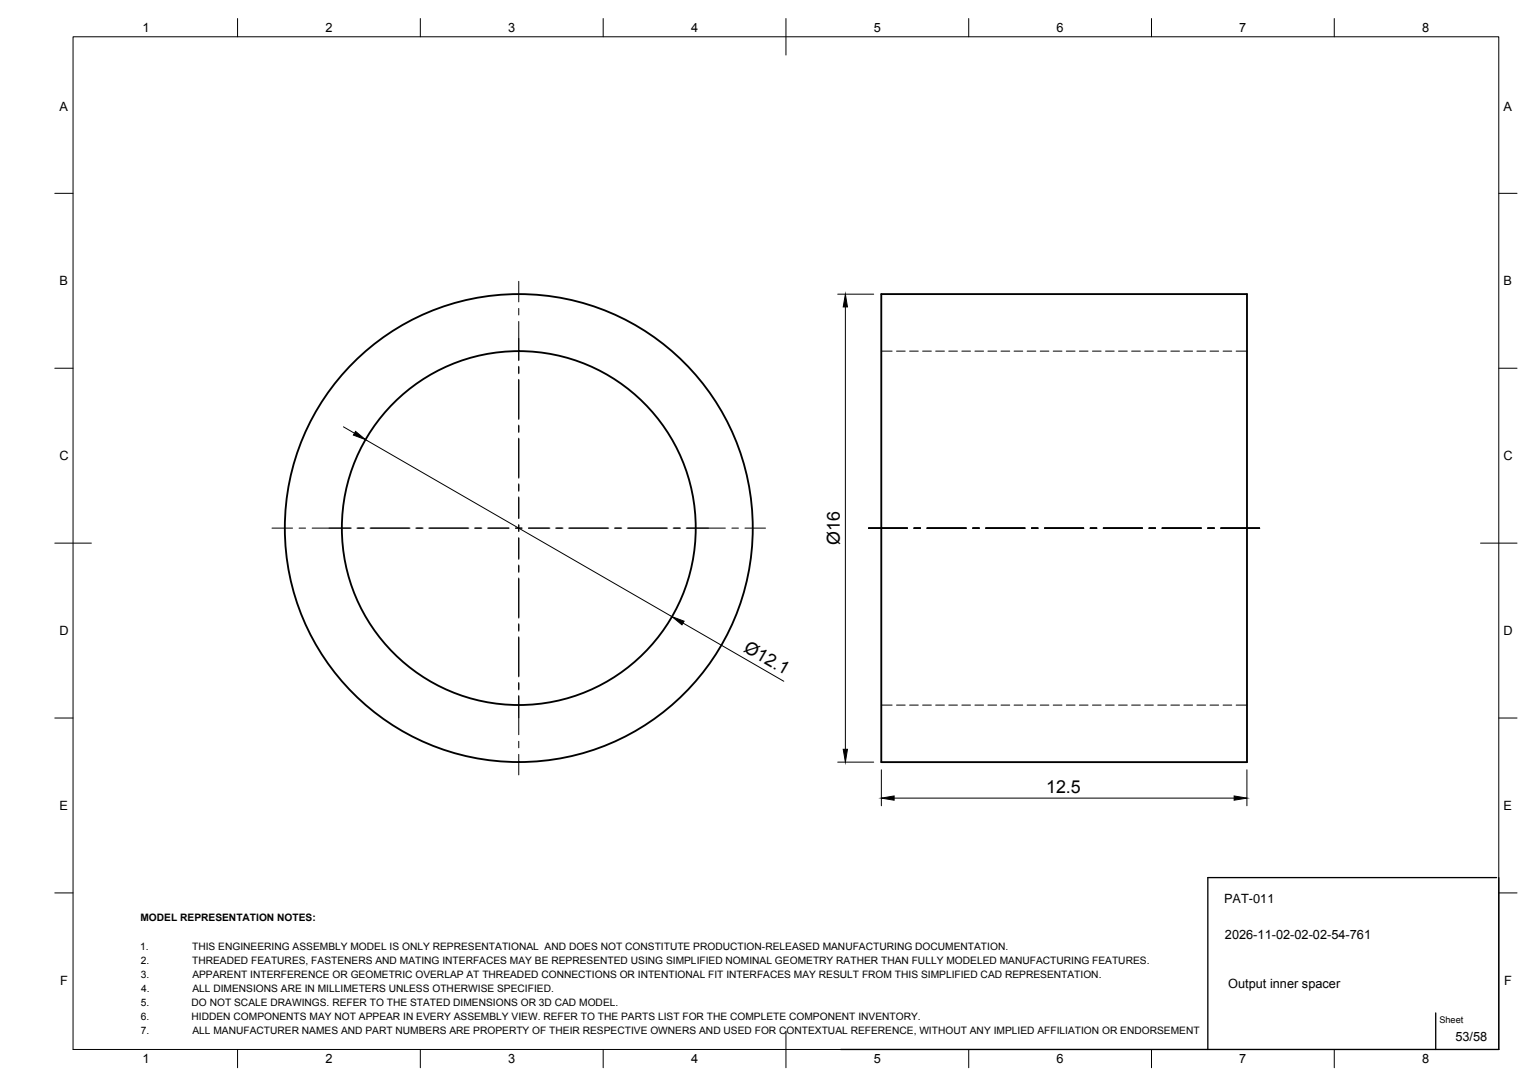
ISO-10303-21;
HEADER;
/* Generated by software containing ST-Developer
 * from STEP Tools, Inc. (www.steptools.com) 
 */

FILE_DESCRIPTION(
/* description */ ('Belt tension measurement rig'),
/* implementation_level */ '2;1');

FILE_NAME(
/* name */ 'Output inner spacer.step',
/* time_stamp */ '2026-10-28T03:24:44-07:00',
/* author */ (''),
/* organization */ (''),
/* preprocessor_version */ 'ST-DEVELOPER v20.2',
/* originating_system */ 'Autodesk Translation Framework v15.17.0.0',
/* authorisation */ '');

FILE_SCHEMA (('AUTOMOTIVE_DESIGN { 1 0 10303 214 3 1 1 }'));
ENDSEC;

DATA;
#10=MECHANICAL_DESIGN_GEOMETRIC_PRESENTATION_REPRESENTATION('',(#752),#23587);
#627=SHAPE_REPRESENTATION_RELATIONSHIP('SRR','None',#23878,#682);
#682=ADVANCED_BREP_SHAPE_REPRESENTATION('',(#820),#23576);
#752=STYLED_ITEM('',(#24204),#820);
#820=MANIFOLD_SOLID_BREP('Body1',#12259);
#1009=FACE_BOUND('',#2779,.T.);
#1010=FACE_BOUND('',#2781,.T.);
#1304=PLANE('',#14039);
#1305=PLANE('',#14040);
#1892=FACE_OUTER_BOUND('',#2776,.T.);
#1893=FACE_OUTER_BOUND('',#2777,.T.);
#1894=FACE_OUTER_BOUND('',#2778,.T.);
#1895=FACE_OUTER_BOUND('',#2780,.T.);
#2776=EDGE_LOOP('',(#10348,#10349,#10350,#10351));
#2777=EDGE_LOOP('',(#10352,#10353,#10354,#10355));
#2778=EDGE_LOOP('',(#10356));
#2779=EDGE_LOOP('',(#10357));
#2780=EDGE_LOOP('',(#10358));
#2781=EDGE_LOOP('',(#10359));
#3561=LINE('',#22187,#4312);
#3562=LINE('',#22193,#4313);
#4312=VECTOR('',#17428,0.605);
#4313=VECTOR('',#17435,0.800000000000001);
#5020=CIRCLE('',#14034,0.605);
#5021=CIRCLE('',#14035,0.605);
#5022=CIRCLE('',#14037,0.800000000000001);
#5023=CIRCLE('',#14038,0.800000000000001);
#6057=VERTEX_POINT('',#22184);
#6058=VERTEX_POINT('',#22186);
#6059=VERTEX_POINT('',#22190);
#6060=VERTEX_POINT('',#22192);
#7533=EDGE_CURVE('',#6057,#6057,#5020,.T.);
#7534=EDGE_CURVE('',#6057,#6058,#3561,.T.);
#7535=EDGE_CURVE('',#6058,#6058,#5021,.T.);
#7536=EDGE_CURVE('',#6059,#6059,#5022,.T.);
#7537=EDGE_CURVE('',#6059,#6060,#3562,.T.);
#7538=EDGE_CURVE('',#6060,#6060,#5023,.T.);
#10348=ORIENTED_EDGE('',*,*,#7533,.F.);
#10349=ORIENTED_EDGE('',*,*,#7534,.T.);
#10350=ORIENTED_EDGE('',*,*,#7535,.T.);
#10351=ORIENTED_EDGE('',*,*,#7534,.F.);
#10352=ORIENTED_EDGE('',*,*,#7536,.F.);
#10353=ORIENTED_EDGE('',*,*,#7537,.T.);
#10354=ORIENTED_EDGE('',*,*,#7538,.T.);
#10355=ORIENTED_EDGE('',*,*,#7537,.F.);
#10356=ORIENTED_EDGE('',*,*,#7536,.T.);
#10357=ORIENTED_EDGE('',*,*,#7533,.T.);
#10358=ORIENTED_EDGE('',*,*,#7538,.F.);
#10359=ORIENTED_EDGE('',*,*,#7535,.F.);
#11383=CYLINDRICAL_SURFACE('',#14033,0.605);
#11384=CYLINDRICAL_SURFACE('',#14036,0.800000000000001);
#12033=ADVANCED_FACE('',(#1892),#11383,.F.);
#12034=ADVANCED_FACE('',(#1893),#11384,.T.);
#12035=ADVANCED_FACE('',(#1894,#1009),#1304,.T.);
#12036=ADVANCED_FACE('',(#1895,#1010),#1305,.F.);
#12259=CLOSED_SHELL('',(#12033,#12034,#12035,#12036));
#14032=AXIS2_PLACEMENT_3D('',#22182,#17422,#17423);
#14033=AXIS2_PLACEMENT_3D('',#22183,#17424,#17425);
#14034=AXIS2_PLACEMENT_3D('',#22185,#17426,#17427);
#14035=AXIS2_PLACEMENT_3D('',#22188,#17429,#17430);
#14036=AXIS2_PLACEMENT_3D('',#22189,#17431,#17432);
#14037=AXIS2_PLACEMENT_3D('',#22191,#17433,#17434);
#14038=AXIS2_PLACEMENT_3D('',#22194,#17436,#17437);
#14039=AXIS2_PLACEMENT_3D('',#22195,#17438,#17439);
#14040=AXIS2_PLACEMENT_3D('',#22196,#17440,#17441);
#17422=DIRECTION('axis',(0.,0.,1.));
#17423=DIRECTION('refdir',(1.,0.,0.));
#17424=DIRECTION('center_axis',(0.,1.,0.));
#17425=DIRECTION('ref_axis',(1.,0.,0.));
#17426=DIRECTION('center_axis',(0.,-1.,0.));
#17427=DIRECTION('ref_axis',(1.,0.,0.));
#17428=DIRECTION('',(0.,-1.,0.));
#17429=DIRECTION('center_axis',(0.,-1.,0.));
#17430=DIRECTION('ref_axis',(1.,0.,0.));
#17431=DIRECTION('center_axis',(0.,1.,0.));
#17432=DIRECTION('ref_axis',(1.,0.,0.));
#17433=DIRECTION('center_axis',(0.,1.,0.));
#17434=DIRECTION('ref_axis',(1.,0.,0.));
#17435=DIRECTION('',(0.,-1.,0.));
#17436=DIRECTION('center_axis',(0.,1.,0.));
#17437=DIRECTION('ref_axis',(1.,0.,0.));
#17438=DIRECTION('center_axis',(0.,1.,0.));
#17439=DIRECTION('ref_axis',(1.,0.,0.));
#17440=DIRECTION('center_axis',(0.,1.,0.));
#17441=DIRECTION('ref_axis',(1.,0.,0.));
#22182=CARTESIAN_POINT('',(0.,0.,0.));
#22183=CARTESIAN_POINT('Origin',(10.,-2.65,7.));
#22184=CARTESIAN_POINT('',(9.395,-1.4,7.));
#22185=CARTESIAN_POINT('Origin',(10.,-1.4,7.));
#22186=CARTESIAN_POINT('',(9.395,-2.65,7.));
#22187=CARTESIAN_POINT('',(9.395,-2.65,7.));
#22188=CARTESIAN_POINT('Origin',(10.,-2.65,7.));
#22189=CARTESIAN_POINT('Origin',(10.,-2.65,7.));
#22190=CARTESIAN_POINT('',(9.2,-1.4,7.));
#22191=CARTESIAN_POINT('Origin',(10.,-1.4,7.));
#22192=CARTESIAN_POINT('',(9.2,-2.65,7.));
#22193=CARTESIAN_POINT('',(9.2,-2.65,7.));
#22194=CARTESIAN_POINT('Origin',(10.,-2.65,7.));
#22195=CARTESIAN_POINT('Origin',(10.,-1.4,7.));
#22196=CARTESIAN_POINT('Origin',(10.,-2.65,7.));
#23511=UNCERTAINTY_MEASURE_WITH_UNIT(LENGTH_MEASURE(0.001),#23588,
'DISTANCE_ACCURACY_VALUE',
'Maximum model space distance between geometric entities at asserted c
onnectivities');
#23522=UNCERTAINTY_MEASURE_WITH_UNIT(LENGTH_MEASURE(0.001),#23588,
'DISTANCE_ACCURACY_VALUE',
'Maximum model space distance between geometric entities at asserted c
onnectivities');
#23576=(
GEOMETRIC_REPRESENTATION_CONTEXT(3)
GLOBAL_UNCERTAINTY_ASSIGNED_CONTEXT((#23511))
GLOBAL_UNIT_ASSIGNED_CONTEXT((#23588,#23590,#23591))
REPRESENTATION_CONTEXT('','3D')
);
#23587=(
GEOMETRIC_REPRESENTATION_CONTEXT(3)
GLOBAL_UNCERTAINTY_ASSIGNED_CONTEXT((#23522))
GLOBAL_UNIT_ASSIGNED_CONTEXT((#23588,#23590,#23591))
REPRESENTATION_CONTEXT('','3D')
);
#23588=(
LENGTH_UNIT()
NAMED_UNIT(*)
SI_UNIT(.CENTI.,.METRE.)
);
#23590=(
NAMED_UNIT(*)
PLANE_ANGLE_UNIT()
SI_UNIT($,.RADIAN.)
);
#23591=(
NAMED_UNIT(*)
SI_UNIT($,.STERADIAN.)
SOLID_ANGLE_UNIT()
);
#23645=SHAPE_DEFINITION_REPRESENTATION(#23722,#23878);
#23722=PRODUCT_DEFINITION_SHAPE('',$,#23943);
#23878=SHAPE_REPRESENTATION('',(#14032),#23576);
#23889=PRODUCT_DEFINITION_CONTEXT('part definition',#24083,'design');
#23943=PRODUCT_DEFINITION('Output inner spacer','Output inner spacer',#24007,
#23889);
#24007=PRODUCT_DEFINITION_FORMATION('',$,#24138);
#24083=APPLICATION_CONTEXT(
'Core Data for Automotive Mechanical Design Process');
#24084=PRODUCT_CONTEXT('part definition',#24083,'mechanical');
#24138=PRODUCT('Output inner spacer','Output inner spacer',
'Output inner spacer',(#24084));
#24198=COLOUR_RGB('Sky Blue',0.24,0.69,0.87);
#24199=FILL_AREA_STYLE_COLOUR('',#24198);
#24200=FILL_AREA_STYLE('',(#24199));
#24201=SURFACE_STYLE_FILL_AREA(#24200);
#24202=SURFACE_SIDE_STYLE('',(#24201));
#24203=SURFACE_STYLE_USAGE(.BOTH.,#24202);
#24204=PRESENTATION_STYLE_ASSIGNMENT((#24203));
ENDSEC;
END-ISO-10303-21;
